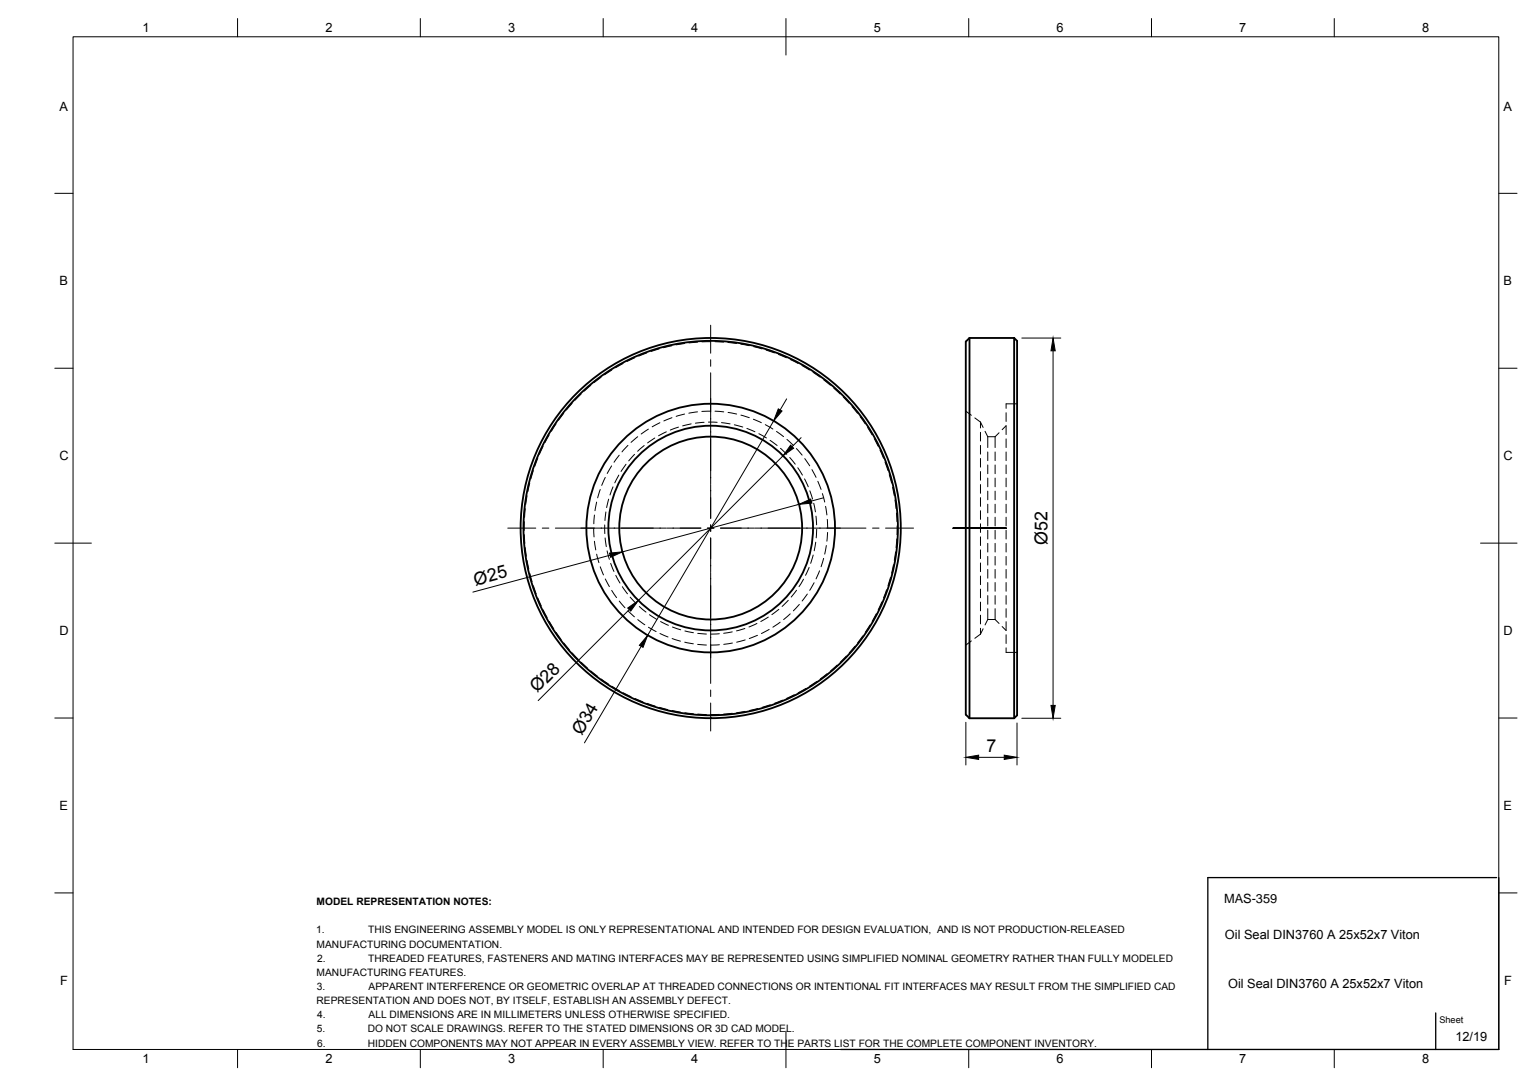
ISO-10303-21;
HEADER;
/* Generated by software containing ST-Developer
 * from STEP Tools, Inc. (www.steptools.com) 
 */

FILE_DESCRIPTION(
/* description */ (''),
/* implementation_level */ '2;1');

FILE_NAME(
/* name */ 'Oil Seal DIN3760 A 25x52x7 Viton.step',
/* time_stamp */ '2026-10-15T14:25:16-07:00',
/* author */ (''),
/* organization */ (''),
/* preprocessor_version */ 'ST-DEVELOPER v20.2',
/* originating_system */ 'Autodesk Translation Framework v15.15.0.0',
/* authorisation */ '');

FILE_SCHEMA (('AUTOMOTIVE_DESIGN { 1 0 10303 214 3 1 1 }'));
ENDSEC;

DATA;
#10=MECHANICAL_DESIGN_GEOMETRIC_PRESENTATION_REPRESENTATION('',(#329),#86429);
#293=SHAPE_REPRESENTATION_RELATIONSHIP('SRR','None',#86508,#311);
#311=ADVANCED_BREP_SHAPE_REPRESENTATION('',(#347),#86417);
#329=STYLED_ITEM('',(#86607),#347);
#347=MANIFOLD_SOLID_BREP('Body1',#15619);
#1303=CONICAL_SURFACE('',#16863,2.575,0.785398163397451);
#1304=CONICAL_SURFACE('',#16867,2.58,0.785398163397448);
#1305=CONICAL_SURFACE('',#16875,1.325,0.785398163397448);
#1306=CONICAL_SURFACE('',#16879,1.35,1.10714871779409);
#1307=CONICAL_SURFACE('',#16881,1.525,0.643501108793285);
#1513=CYLINDRICAL_SURFACE('',#16865,2.6);
#1514=CYLINDRICAL_SURFACE('',#16871,1.7);
#1515=CYLINDRICAL_SURFACE('',#16877,1.25);
#1712=FACE_BOUND('',#4017,.T.);
#1713=FACE_BOUND('',#4022,.T.);
#1714=FACE_BOUND('',#4025,.T.);
#2216=CIRCLE('',#16861,2.55);
#2217=CIRCLE('',#16862,1.6);
#2218=CIRCLE('',#16864,2.6);
#2219=CIRCLE('',#16866,2.6);
#2220=CIRCLE('',#16868,2.56);
#2221=CIRCLE('',#16870,1.7);
#2222=CIRCLE('',#16872,1.7);
#2223=CIRCLE('',#16874,1.4);
#2224=CIRCLE('',#16876,1.25);
#2225=CIRCLE('',#16878,1.25);
#2226=CIRCLE('',#16880,1.45);
#3034=FACE_OUTER_BOUND('',#4016,.T.);
#3035=FACE_OUTER_BOUND('',#4018,.T.);
#3036=FACE_OUTER_BOUND('',#4019,.T.);
#3037=FACE_OUTER_BOUND('',#4020,.T.);
#3038=FACE_OUTER_BOUND('',#4021,.T.);
#3039=FACE_OUTER_BOUND('',#4023,.T.);
#3040=FACE_OUTER_BOUND('',#4024,.T.);
#3041=FACE_OUTER_BOUND('',#4026,.T.);
#3042=FACE_OUTER_BOUND('',#4027,.T.);
#3043=FACE_OUTER_BOUND('',#4028,.T.);
#3044=FACE_OUTER_BOUND('',#4029,.T.);
#4016=EDGE_LOOP('',(#13239));
#4017=EDGE_LOOP('',(#13240));
#4018=EDGE_LOOP('',(#13241,#13242,#13243,#13244));
#4019=EDGE_LOOP('',(#13245,#13246,#13247,#13248));
#4020=EDGE_LOOP('',(#13249,#13250,#13251,#13252));
#4021=EDGE_LOOP('',(#13253));
#4022=EDGE_LOOP('',(#13254));
#4023=EDGE_LOOP('',(#13255,#13256,#13257,#13258));
#4024=EDGE_LOOP('',(#13259));
#4025=EDGE_LOOP('',(#13260));
#4026=EDGE_LOOP('',(#13261,#13262,#13263,#13264));
#4027=EDGE_LOOP('',(#13265,#13266,#13267,#13268));
#4028=EDGE_LOOP('',(#13269,#13270,#13271,#13272));
#4029=EDGE_LOOP('',(#13273,#13274,#13275,#13276));
#4968=LINE('',#63188,#5828);
#4969=LINE('',#63192,#5829);
#4970=LINE('',#63195,#5830);
#4971=LINE('',#63203,#5831);
#4972=LINE('',#63210,#5832);
#4973=LINE('',#63214,#5833);
#4974=LINE('',#63217,#5834);
#4975=LINE('',#63220,#5835);
#5828=VECTOR('',#20043,2.575);
#5829=VECTOR('',#20048,2.6);
#5830=VECTOR('',#20051,2.58);
#5831=VECTOR('',#20062,1.7);
#5832=VECTOR('',#20071,1.325);
#5833=VECTOR('',#20076,1.25);
#5834=VECTOR('',#20079,1.35);
#5835=VECTOR('',#20084,1.525);
#7108=VERTEX_POINT('',#63181);
#7109=VERTEX_POINT('',#63183);
#7110=VERTEX_POINT('',#63186);
#7111=VERTEX_POINT('',#63190);
#7112=VERTEX_POINT('',#63194);
#7113=VERTEX_POINT('',#63198);
#7114=VERTEX_POINT('',#63201);
#7115=VERTEX_POINT('',#63205);
#7116=VERTEX_POINT('',#63208);
#7117=VERTEX_POINT('',#63212);
#7118=VERTEX_POINT('',#63216);
#9241=EDGE_CURVE('',#7108,#7108,#2216,.T.);
#9242=EDGE_CURVE('',#7109,#7109,#2217,.T.);
#9243=EDGE_CURVE('',#7110,#7110,#2218,.T.);
#9244=EDGE_CURVE('',#7110,#7108,#4968,.T.);
#9245=EDGE_CURVE('',#7111,#7111,#2219,.T.);
#9246=EDGE_CURVE('',#7111,#7110,#4969,.T.);
#9247=EDGE_CURVE('',#7111,#7112,#4970,.T.);
#9248=EDGE_CURVE('',#7112,#7112,#2220,.T.);
#9249=EDGE_CURVE('',#7113,#7113,#2221,.T.);
#9250=EDGE_CURVE('',#7114,#7114,#2222,.T.);
#9251=EDGE_CURVE('',#7114,#7113,#4971,.T.);
#9252=EDGE_CURVE('',#7115,#7115,#2223,.T.);
#9253=EDGE_CURVE('',#7116,#7116,#2224,.T.);
#9254=EDGE_CURVE('',#7116,#7115,#4972,.T.);
#9255=EDGE_CURVE('',#7117,#7117,#2225,.T.);
#9256=EDGE_CURVE('',#7117,#7116,#4973,.T.);
#9257=EDGE_CURVE('',#7117,#7118,#4974,.T.);
#9258=EDGE_CURVE('',#7118,#7118,#2226,.T.);
#9259=EDGE_CURVE('',#7118,#7109,#4975,.T.);
#13239=ORIENTED_EDGE('',*,*,#9241,.F.);
#13240=ORIENTED_EDGE('',*,*,#9242,.T.);
#13241=ORIENTED_EDGE('',*,*,#9243,.F.);
#13242=ORIENTED_EDGE('',*,*,#9244,.T.);
#13243=ORIENTED_EDGE('',*,*,#9241,.T.);
#13244=ORIENTED_EDGE('',*,*,#9244,.F.);
#13245=ORIENTED_EDGE('',*,*,#9245,.F.);
#13246=ORIENTED_EDGE('',*,*,#9246,.T.);
#13247=ORIENTED_EDGE('',*,*,#9243,.T.);
#13248=ORIENTED_EDGE('',*,*,#9246,.F.);
#13249=ORIENTED_EDGE('',*,*,#9245,.T.);
#13250=ORIENTED_EDGE('',*,*,#9247,.T.);
#13251=ORIENTED_EDGE('',*,*,#9248,.F.);
#13252=ORIENTED_EDGE('',*,*,#9247,.F.);
#13253=ORIENTED_EDGE('',*,*,#9248,.T.);
#13254=ORIENTED_EDGE('',*,*,#9249,.F.);
#13255=ORIENTED_EDGE('',*,*,#9250,.F.);
#13256=ORIENTED_EDGE('',*,*,#9251,.T.);
#13257=ORIENTED_EDGE('',*,*,#9249,.T.);
#13258=ORIENTED_EDGE('',*,*,#9251,.F.);
#13259=ORIENTED_EDGE('',*,*,#9250,.T.);
#13260=ORIENTED_EDGE('',*,*,#9252,.F.);
#13261=ORIENTED_EDGE('',*,*,#9253,.F.);
#13262=ORIENTED_EDGE('',*,*,#9254,.T.);
#13263=ORIENTED_EDGE('',*,*,#9252,.T.);
#13264=ORIENTED_EDGE('',*,*,#9254,.F.);
#13265=ORIENTED_EDGE('',*,*,#9255,.F.);
#13266=ORIENTED_EDGE('',*,*,#9256,.T.);
#13267=ORIENTED_EDGE('',*,*,#9253,.T.);
#13268=ORIENTED_EDGE('',*,*,#9256,.F.);
#13269=ORIENTED_EDGE('',*,*,#9255,.T.);
#13270=ORIENTED_EDGE('',*,*,#9257,.T.);
#13271=ORIENTED_EDGE('',*,*,#9258,.F.);
#13272=ORIENTED_EDGE('',*,*,#9257,.F.);
#13273=ORIENTED_EDGE('',*,*,#9258,.T.);
#13274=ORIENTED_EDGE('',*,*,#9259,.T.);
#13275=ORIENTED_EDGE('',*,*,#9242,.F.);
#13276=ORIENTED_EDGE('',*,*,#9259,.F.);
#14665=PLANE('',#16860);
#14666=PLANE('',#16869);
#14667=PLANE('',#16873);
#15390=ADVANCED_FACE('',(#3034,#1712),#14665,.T.);
#15391=ADVANCED_FACE('',(#3035),#1303,.T.);
#15392=ADVANCED_FACE('',(#3036),#1513,.T.);
#15393=ADVANCED_FACE('',(#3037),#1304,.T.);
#15394=ADVANCED_FACE('',(#3038,#1713),#14666,.T.);
#15395=ADVANCED_FACE('',(#3039),#1514,.F.);
#15396=ADVANCED_FACE('',(#3040,#1714),#14667,.T.);
#15397=ADVANCED_FACE('',(#3041),#1305,.F.);
#15398=ADVANCED_FACE('',(#3042),#1515,.F.);
#15399=ADVANCED_FACE('',(#3043),#1306,.F.);
#15400=ADVANCED_FACE('',(#3044),#1307,.F.);
#15619=CLOSED_SHELL('',(#15390,#15391,#15392,#15393,#15394,#15395,#15396,
#15397,#15398,#15399,#15400));
#16859=AXIS2_PLACEMENT_3D('',#63179,#20031,#20032);
#16860=AXIS2_PLACEMENT_3D('',#63180,#20033,#20034);
#16861=AXIS2_PLACEMENT_3D('',#63182,#20035,#20036);
#16862=AXIS2_PLACEMENT_3D('',#63184,#20037,#20038);
#16863=AXIS2_PLACEMENT_3D('',#63185,#20039,#20040);
#16864=AXIS2_PLACEMENT_3D('',#63187,#20041,#20042);
#16865=AXIS2_PLACEMENT_3D('',#63189,#20044,#20045);
#16866=AXIS2_PLACEMENT_3D('',#63191,#20046,#20047);
#16867=AXIS2_PLACEMENT_3D('',#63193,#20049,#20050);
#16868=AXIS2_PLACEMENT_3D('',#63196,#20052,#20053);
#16869=AXIS2_PLACEMENT_3D('',#63197,#20054,#20055);
#16870=AXIS2_PLACEMENT_3D('',#63199,#20056,#20057);
#16871=AXIS2_PLACEMENT_3D('',#63200,#20058,#20059);
#16872=AXIS2_PLACEMENT_3D('',#63202,#20060,#20061);
#16873=AXIS2_PLACEMENT_3D('',#63204,#20063,#20064);
#16874=AXIS2_PLACEMENT_3D('',#63206,#20065,#20066);
#16875=AXIS2_PLACEMENT_3D('',#63207,#20067,#20068);
#16876=AXIS2_PLACEMENT_3D('',#63209,#20069,#20070);
#16877=AXIS2_PLACEMENT_3D('',#63211,#20072,#20073);
#16878=AXIS2_PLACEMENT_3D('',#63213,#20074,#20075);
#16879=AXIS2_PLACEMENT_3D('',#63215,#20077,#20078);
#16880=AXIS2_PLACEMENT_3D('',#63218,#20080,#20081);
#16881=AXIS2_PLACEMENT_3D('',#63219,#20082,#20083);
#20031=DIRECTION('axis',(0.,0.,1.));
#20032=DIRECTION('refdir',(1.,0.,0.));
#20033=DIRECTION('center_axis',(0.,0.,-1.));
#20034=DIRECTION('ref_axis',(-1.,0.,0.));
#20035=DIRECTION('center_axis',(0.,0.,1.));
#20036=DIRECTION('ref_axis',(1.,0.,0.));
#20037=DIRECTION('center_axis',(0.,0.,1.));
#20038=DIRECTION('ref_axis',(1.,0.,0.));
#20039=DIRECTION('center_axis',(0.,0.,1.));
#20040=DIRECTION('ref_axis',(1.,0.,0.));
#20041=DIRECTION('center_axis',(0.,0.,1.));
#20042=DIRECTION('ref_axis',(1.,0.,0.));
#20043=DIRECTION('',(0.707106781186549,8.65956056235496E-17,-0.707106781186546));
#20044=DIRECTION('center_axis',(0.,0.,1.));
#20045=DIRECTION('ref_axis',(1.,0.,0.));
#20046=DIRECTION('center_axis',(0.,0.,1.));
#20047=DIRECTION('ref_axis',(1.,0.,0.));
#20048=DIRECTION('',(0.,0.,-1.));
#20049=DIRECTION('center_axis',(0.,0.,-1.));
#20050=DIRECTION('ref_axis',(1.,0.,0.));
#20051=DIRECTION('',(0.707106781186547,-8.65956056235493E-17,0.707106781186548));
#20052=DIRECTION('center_axis',(0.,0.,1.));
#20053=DIRECTION('ref_axis',(1.,0.,0.));
#20054=DIRECTION('center_axis',(0.,0.,1.));
#20055=DIRECTION('ref_axis',(1.,0.,0.));
#20056=DIRECTION('center_axis',(0.,0.,1.));
#20057=DIRECTION('ref_axis',(1.,0.,0.));
#20058=DIRECTION('center_axis',(0.,0.,1.));
#20059=DIRECTION('ref_axis',(1.,0.,0.));
#20060=DIRECTION('center_axis',(0.,0.,1.));
#20061=DIRECTION('ref_axis',(1.,0.,0.));
#20062=DIRECTION('',(0.,0.,1.));
#20063=DIRECTION('center_axis',(0.,0.,1.));
#20064=DIRECTION('ref_axis',(1.,0.,0.));
#20065=DIRECTION('center_axis',(0.,0.,1.));
#20066=DIRECTION('ref_axis',(1.,0.,0.));
#20067=DIRECTION('center_axis',(0.,0.,1.));
#20068=DIRECTION('ref_axis',(1.,0.,0.));
#20069=DIRECTION('center_axis',(0.,0.,1.));
#20070=DIRECTION('ref_axis',(1.,0.,0.));
#20071=DIRECTION('',(-0.707106781186547,-8.65956056235493E-17,0.707106781186548));
#20072=DIRECTION('center_axis',(0.,0.,1.));
#20073=DIRECTION('ref_axis',(1.,0.,0.));
#20074=DIRECTION('center_axis',(0.,0.,1.));
#20075=DIRECTION('ref_axis',(1.,0.,0.));
#20076=DIRECTION('',(0.,0.,1.));
#20077=DIRECTION('center_axis',(0.,0.,-1.));
#20078=DIRECTION('ref_axis',(1.,0.,0.));
#20079=DIRECTION('',(-0.894427190999916,1.09535739652841E-16,-0.447213595499958));
#20080=DIRECTION('center_axis',(0.,0.,1.));
#20081=DIRECTION('ref_axis',(1.,0.,0.));
#20082=DIRECTION('center_axis',(0.,0.,-1.));
#20083=DIRECTION('ref_axis',(1.,0.,0.));
#20084=DIRECTION('',(-0.600000000000001,7.34788079488413E-17,-0.8));
#63179=CARTESIAN_POINT('',(0.,0.,0.));
#63180=CARTESIAN_POINT('Origin',(2.55,0.,0.));
#63181=CARTESIAN_POINT('',(-2.55,-3.12284933782575E-16,-1.17961196366423E-16));
#63182=CARTESIAN_POINT('Origin',(0.,0.,0.));
#63183=CARTESIAN_POINT('',(-1.6,-1.95943487863577E-16,-2.77555756156289E-17));
#63184=CARTESIAN_POINT('Origin',(0.,0.,0.));
#63185=CARTESIAN_POINT('Origin',(0.,0.,0.025));
#63186=CARTESIAN_POINT('',(-2.6,-3.18408167778312E-16,0.0499999999999999));
#63187=CARTESIAN_POINT('Origin',(0.,0.,0.05));
#63188=CARTESIAN_POINT('',(-2.575,-3.15346550780443E-16,0.025));
#63189=CARTESIAN_POINT('Origin',(0.,0.,0.355));
#63190=CARTESIAN_POINT('',(-2.6,-3.18408167778312E-16,0.66));
#63191=CARTESIAN_POINT('Origin',(0.,0.,0.66));
#63192=CARTESIAN_POINT('',(-2.6,-3.18408167778312E-16,0.355));
#63193=CARTESIAN_POINT('Origin',(0.,0.,0.68));
#63194=CARTESIAN_POINT('',(-2.56,-3.13509580581722E-16,0.7));
#63195=CARTESIAN_POINT('',(-2.58,3.15958874180017E-16,0.68));
#63196=CARTESIAN_POINT('Origin',(0.,0.,0.7));
#63197=CARTESIAN_POINT('Origin',(1.7,0.,0.7));
#63198=CARTESIAN_POINT('',(-1.7,-2.0818995585505E-16,0.7));
#63199=CARTESIAN_POINT('Origin',(0.,0.,0.7));
#63200=CARTESIAN_POINT('Origin',(0.,0.,0.625));
#63201=CARTESIAN_POINT('',(-1.7,-2.0818995585505E-16,0.55));
#63202=CARTESIAN_POINT('Origin',(0.,0.,0.55));
#63203=CARTESIAN_POINT('',(-1.7,-2.0818995585505E-16,0.625));
#63204=CARTESIAN_POINT('Origin',(1.4,0.,0.55));
#63205=CARTESIAN_POINT('',(-1.4,-1.71450551880629E-16,0.55));
#63206=CARTESIAN_POINT('Origin',(0.,0.,0.55));
#63207=CARTESIAN_POINT('Origin',(0.,0.,0.475));
#63208=CARTESIAN_POINT('',(-1.25,-1.53080849893419E-16,0.4));
#63209=CARTESIAN_POINT('Origin',(0.,0.,0.4));
#63210=CARTESIAN_POINT('',(-1.325,-1.62265700887024E-16,0.475));
#63211=CARTESIAN_POINT('Origin',(0.,0.,0.35));
#63212=CARTESIAN_POINT('',(-1.25,-1.53080849893419E-16,0.3));
#63213=CARTESIAN_POINT('Origin',(0.,0.,0.3));
#63214=CARTESIAN_POINT('',(-1.25,-1.53080849893419E-16,0.35));
#63215=CARTESIAN_POINT('Origin',(0.,0.,0.25));
#63216=CARTESIAN_POINT('',(-1.45,-1.77573785876366E-16,0.2));
#63217=CARTESIAN_POINT('',(-1.35,1.65327317884893E-16,0.25));
#63218=CARTESIAN_POINT('Origin',(0.,0.,0.2));
#63219=CARTESIAN_POINT('Origin',(0.,0.,0.1));
#63220=CARTESIAN_POINT('',(-1.525,1.86758636869971E-16,0.1));
#86397=UNCERTAINTY_MEASURE_WITH_UNIT(LENGTH_MEASURE(0.001),#86430,
'DISTANCE_ACCURACY_VALUE',
'Maximum model space distance between geometric entities at asserted c
onnectivities');
#86409=UNCERTAINTY_MEASURE_WITH_UNIT(LENGTH_MEASURE(0.001),#86430,
'DISTANCE_ACCURACY_VALUE',
'Maximum model space distance between geometric entities at asserted c
onnectivities');
#86417=(
GEOMETRIC_REPRESENTATION_CONTEXT(3)
GLOBAL_UNCERTAINTY_ASSIGNED_CONTEXT((#86397))
GLOBAL_UNIT_ASSIGNED_CONTEXT((#86430,#86432,#86433))
REPRESENTATION_CONTEXT('','3D')
);
#86429=(
GEOMETRIC_REPRESENTATION_CONTEXT(3)
GLOBAL_UNCERTAINTY_ASSIGNED_CONTEXT((#86409))
GLOBAL_UNIT_ASSIGNED_CONTEXT((#86430,#86432,#86433))
REPRESENTATION_CONTEXT('','3D')
);
#86430=(
LENGTH_UNIT()
NAMED_UNIT(*)
SI_UNIT(.CENTI.,.METRE.)
);
#86432=(
NAMED_UNIT(*)
PLANE_ANGLE_UNIT()
SI_UNIT($,.RADIAN.)
);
#86433=(
NAMED_UNIT(*)
SI_UNIT($,.STERADIAN.)
SOLID_ANGLE_UNIT()
);
#86441=SHAPE_DEFINITION_REPRESENTATION(#86460,#86508);
#86460=PRODUCT_DEFINITION_SHAPE('',$,#86528);
#86508=SHAPE_REPRESENTATION('',(#16859),#86417);
#86520=PRODUCT_DEFINITION_CONTEXT('part definition',#86579,'design');
#86528=PRODUCT_DEFINITION('Oil Seal DIN3760 A 25x52x7 Viton',
'Oil Seal DIN3760 A 25x52x7 Viton',#86547,#86520);
#86547=PRODUCT_DEFINITION_FORMATION('',$,#86588);
#86579=APPLICATION_CONTEXT(
'Core Data for Automotive Mechanical Design Process');
#86580=PRODUCT_CONTEXT('part definition',#86579,'mechanical');
#86588=PRODUCT('Oil Seal DIN3760 A 25x52x7 Viton',
'Oil Seal DIN3760 A 25x52x7 Viton',$,(#86580));
#86607=PRESENTATION_STYLE_ASSIGNMENT((#86625));
#86625=SURFACE_STYLE_USAGE(.BOTH.,#86643);
#86643=SURFACE_SIDE_STYLE('',(#86661));
#86661=SURFACE_STYLE_FILL_AREA(#86679);
#86679=FILL_AREA_STYLE('Opaque(52,52,56)',(#86697));
#86697=FILL_AREA_STYLE_COLOUR('Opaque(52,52,56)',#86715);
#86715=COLOUR_RGB('Opaque(52,52,56)', 0.09019608, 0.27058824, 0.51372549);
ENDSEC;
END-ISO-10303-21;
